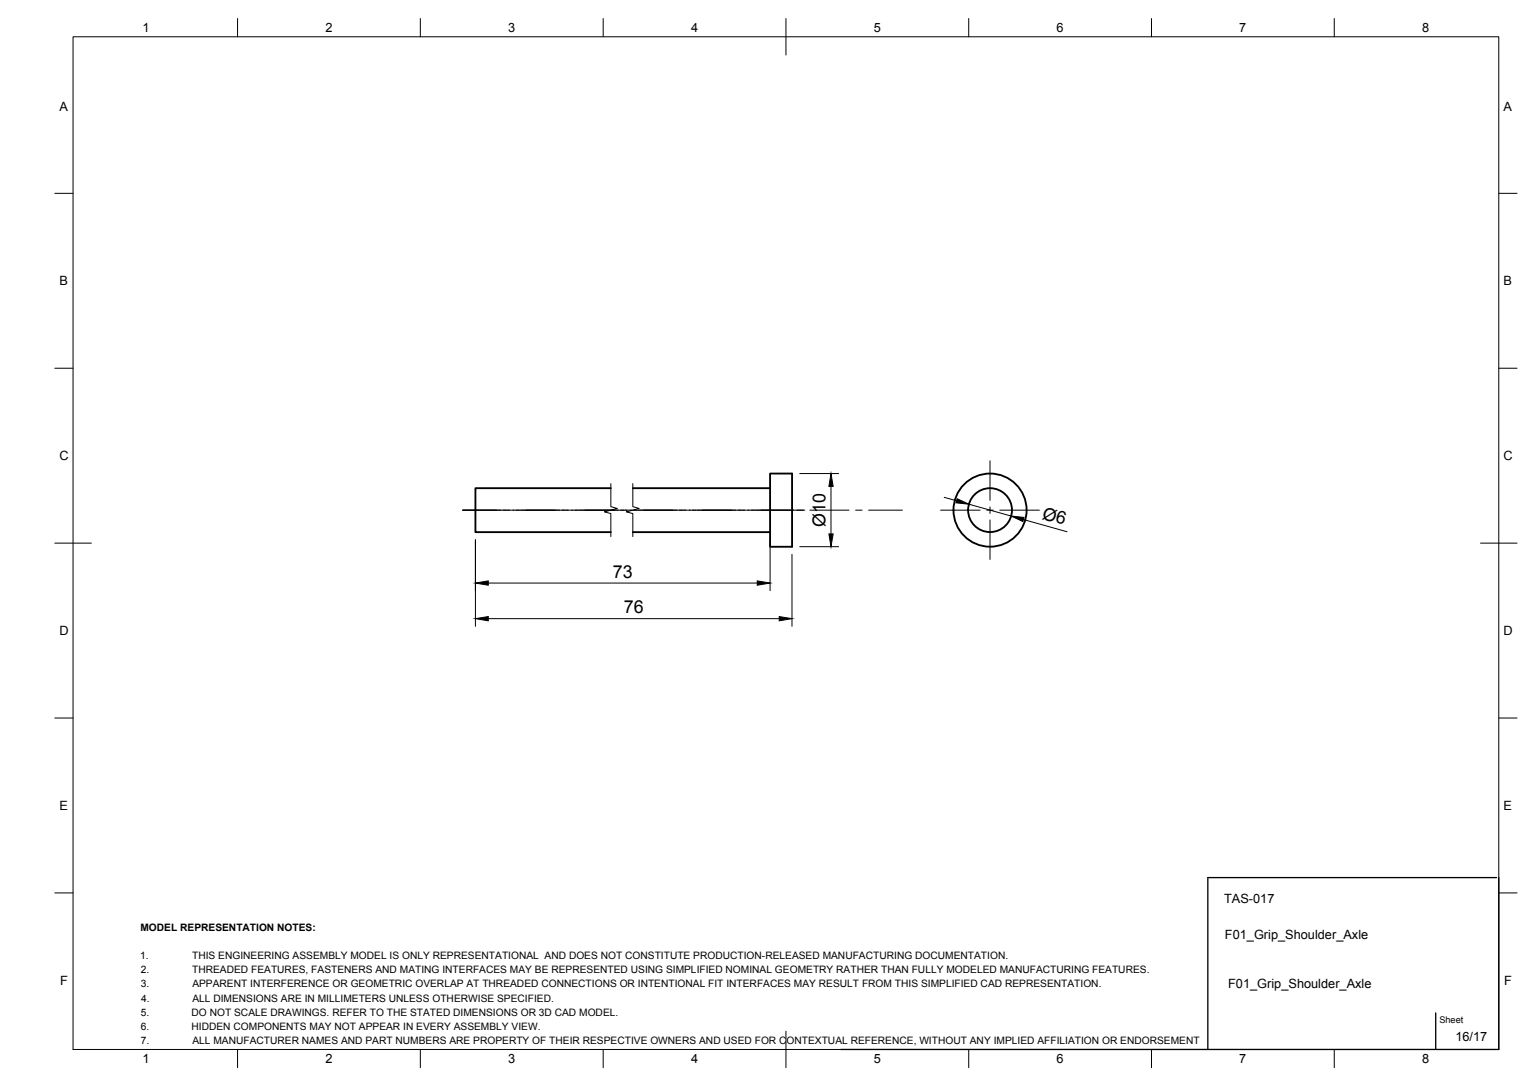
ISO-10303-21;
HEADER;
/* Generated by software containing ST-Developer
 * from STEP Tools, Inc. (www.steptools.com) 
 */

FILE_DESCRIPTION(
/* description */ ('STEP AP203'),
/* implementation_level */ '2;1');

FILE_NAME(
/* name */ 'F01_Grip_Shoulder_Axle.step',
/* time_stamp */ '2026-11-15T15:04:01-08:00',
/* author */ (''),
/* organization */ (''),
/* preprocessor_version */ 'ST-DEVELOPER v20.2',
/* originating_system */ 'Autodesk Translation Framework v15.17.0.0',
/* authorisation */ '');

FILE_SCHEMA (('AUTOMOTIVE_DESIGN { 1 0 10303 214 3 1 1 }'));
ENDSEC;

DATA;
#10=MECHANICAL_DESIGN_GEOMETRIC_PRESENTATION_REPRESENTATION('',(#301),#16598);
#223=SHAPE_REPRESENTATION_RELATIONSHIP('SRR','None',#16717,#247);
#247=ADVANCED_BREP_SHAPE_REPRESENTATION('',(#271),#16593);
#271=MANIFOLD_SOLID_BREP('Body1',#9806);
#301=STYLED_ITEM('',(#16829),#271);
#421=FACE_BOUND('',#2085,.T.);
#871=PLANE('',#10822);
#872=PLANE('',#10823);
#873=PLANE('',#10824);
#1414=FACE_OUTER_BOUND('',#2080,.T.);
#1415=FACE_OUTER_BOUND('',#2081,.T.);
#1416=FACE_OUTER_BOUND('',#2082,.T.);
#1417=FACE_OUTER_BOUND('',#2083,.T.);
#1418=FACE_OUTER_BOUND('',#2084,.T.);
#2080=EDGE_LOOP('',(#8977,#8978,#8979,#8980));
#2081=EDGE_LOOP('',(#8981,#8982,#8983,#8984));
#2082=EDGE_LOOP('',(#8985));
#2083=EDGE_LOOP('',(#8986));
#2084=EDGE_LOOP('',(#8987));
#2085=EDGE_LOOP('',(#8988));
#3104=LINE('',#16295,#4152);
#3105=LINE('',#16301,#4153);
#4152=VECTOR('',#13380,5.);
#4153=VECTOR('',#13387,3.);
#4439=CIRCLE('',#10817,5.);
#4440=CIRCLE('',#10818,5.);
#4441=CIRCLE('',#10820,3.);
#4442=CIRCLE('',#10821,3.);
#5247=VERTEX_POINT('',#16292);
#5248=VERTEX_POINT('',#16294);
#5249=VERTEX_POINT('',#16298);
#5250=VERTEX_POINT('',#16300);
#6501=EDGE_CURVE('',#5247,#5247,#4439,.T.);
#6502=EDGE_CURVE('',#5247,#5248,#3104,.T.);
#6503=EDGE_CURVE('',#5248,#5248,#4440,.T.);
#6504=EDGE_CURVE('',#5249,#5249,#4441,.T.);
#6505=EDGE_CURVE('',#5249,#5250,#3105,.T.);
#6506=EDGE_CURVE('',#5250,#5250,#4442,.T.);
#8977=ORIENTED_EDGE('',*,*,#6501,.T.);
#8978=ORIENTED_EDGE('',*,*,#6502,.T.);
#8979=ORIENTED_EDGE('',*,*,#6503,.F.);
#8980=ORIENTED_EDGE('',*,*,#6502,.F.);
#8981=ORIENTED_EDGE('',*,*,#6504,.T.);
#8982=ORIENTED_EDGE('',*,*,#6505,.T.);
#8983=ORIENTED_EDGE('',*,*,#6506,.F.);
#8984=ORIENTED_EDGE('',*,*,#6505,.F.);
#8985=ORIENTED_EDGE('',*,*,#6504,.F.);
#8986=ORIENTED_EDGE('',*,*,#6503,.T.);
#8987=ORIENTED_EDGE('',*,*,#6501,.F.);
#8988=ORIENTED_EDGE('',*,*,#6506,.T.);
#9228=CYLINDRICAL_SURFACE('',#10816,5.);
#9229=CYLINDRICAL_SURFACE('',#10819,3.);
#9739=ADVANCED_FACE('',(#1414),#9228,.T.);
#9740=ADVANCED_FACE('',(#1415),#9229,.T.);
#9741=ADVANCED_FACE('',(#1416),#871,.F.);
#9742=ADVANCED_FACE('',(#1417),#872,.T.);
#9743=ADVANCED_FACE('',(#1418,#421),#873,.F.);
#9806=CLOSED_SHELL('',(#9739,#9740,#9741,#9742,#9743));
#10815=AXIS2_PLACEMENT_3D('',#16290,#13374,#13375);
#10816=AXIS2_PLACEMENT_3D('',#16291,#13376,#13377);
#10817=AXIS2_PLACEMENT_3D('',#16293,#13378,#13379);
#10818=AXIS2_PLACEMENT_3D('',#16296,#13381,#13382);
#10819=AXIS2_PLACEMENT_3D('',#16297,#13383,#13384);
#10820=AXIS2_PLACEMENT_3D('',#16299,#13385,#13386);
#10821=AXIS2_PLACEMENT_3D('',#16302,#13388,#13389);
#10822=AXIS2_PLACEMENT_3D('',#16303,#13390,#13391);
#10823=AXIS2_PLACEMENT_3D('',#16304,#13392,#13393);
#10824=AXIS2_PLACEMENT_3D('',#16305,#13394,#13395);
#13374=DIRECTION('axis',(0.,0.,1.));
#13375=DIRECTION('refdir',(1.,0.,0.));
#13376=DIRECTION('center_axis',(0.,0.,-1.));
#13377=DIRECTION('ref_axis',(-1.,0.,0.));
#13378=DIRECTION('center_axis',(0.,0.,1.));
#13379=DIRECTION('ref_axis',(1.,0.,0.));
#13380=DIRECTION('',(0.,0.,1.));
#13381=DIRECTION('center_axis',(0.,0.,1.));
#13382=DIRECTION('ref_axis',(1.,0.,0.));
#13383=DIRECTION('center_axis',(0.,0.,-1.));
#13384=DIRECTION('ref_axis',(-1.,0.,0.));
#13385=DIRECTION('center_axis',(0.,0.,1.));
#13386=DIRECTION('ref_axis',(1.,0.,0.));
#13387=DIRECTION('',(0.,0.,1.));
#13388=DIRECTION('center_axis',(0.,0.,1.));
#13389=DIRECTION('ref_axis',(1.,0.,0.));
#13390=DIRECTION('center_axis',(0.,0.,1.));
#13391=DIRECTION('ref_axis',(1.,0.,0.));
#13392=DIRECTION('center_axis',(0.,0.,1.));
#13393=DIRECTION('ref_axis',(1.,0.,0.));
#13394=DIRECTION('center_axis',(0.,0.,1.));
#13395=DIRECTION('ref_axis',(1.,0.,0.));
#16290=CARTESIAN_POINT('',(0.,0.,0.));
#16291=CARTESIAN_POINT('Origin',(0.,0.,76.));
#16292=CARTESIAN_POINT('',(5.,-6.12323399573677E-16,73.));
#16293=CARTESIAN_POINT('Origin',(0.,0.,73.));
#16294=CARTESIAN_POINT('',(5.,-6.12323399573677E-16,76.));
#16295=CARTESIAN_POINT('',(5.,-6.12323399573677E-16,76.));
#16296=CARTESIAN_POINT('Origin',(0.,0.,76.));
#16297=CARTESIAN_POINT('Origin',(0.,0.,73.));
#16298=CARTESIAN_POINT('',(3.,-3.67394039744206E-16,0.));
#16299=CARTESIAN_POINT('Origin',(0.,0.,0.));
#16300=CARTESIAN_POINT('',(3.,-3.67394039744206E-16,73.));
#16301=CARTESIAN_POINT('',(3.,-3.67394039744206E-16,73.));
#16302=CARTESIAN_POINT('Origin',(0.,0.,73.));
#16303=CARTESIAN_POINT('Origin',(0.,0.,0.));
#16304=CARTESIAN_POINT('Origin',(0.,0.,76.));
#16305=CARTESIAN_POINT('Origin',(0.,0.,73.));
#16567=UNCERTAINTY_MEASURE_WITH_UNIT(LENGTH_MEASURE(0.01),#16599,
'DISTANCE_ACCURACY_VALUE',
'Maximum model space distance between geometric entities at asserted c
onnectivities');
#16572=UNCERTAINTY_MEASURE_WITH_UNIT(LENGTH_MEASURE(0.01),#16599,
'DISTANCE_ACCURACY_VALUE',
'Maximum model space distance between geometric entities at asserted c
onnectivities');
#16593=(
GEOMETRIC_REPRESENTATION_CONTEXT(3)
GLOBAL_UNCERTAINTY_ASSIGNED_CONTEXT((#16567))
GLOBAL_UNIT_ASSIGNED_CONTEXT((#16599,#16601,#16602))
REPRESENTATION_CONTEXT('','3D')
);
#16598=(
GEOMETRIC_REPRESENTATION_CONTEXT(3)
GLOBAL_UNCERTAINTY_ASSIGNED_CONTEXT((#16572))
GLOBAL_UNIT_ASSIGNED_CONTEXT((#16599,#16601,#16602))
REPRESENTATION_CONTEXT('','3D')
);
#16599=(
LENGTH_UNIT()
NAMED_UNIT(*)
SI_UNIT(.MILLI.,.METRE.)
);
#16601=(
NAMED_UNIT(*)
PLANE_ANGLE_UNIT()
SI_UNIT($,.RADIAN.)
);
#16602=(
NAMED_UNIT(*)
SI_UNIT($,.STERADIAN.)
SOLID_ANGLE_UNIT()
);
#16623=SHAPE_DEFINITION_REPRESENTATION(#16648,#16717);
#16648=PRODUCT_DEFINITION_SHAPE('',$,#16743);
#16717=SHAPE_REPRESENTATION('',(#10815),#16593);
#16722=PRODUCT_DEFINITION_CONTEXT('part definition',#16799,'design');
#16743=PRODUCT_DEFINITION('F01_Grip_Shoulder_Axle',
'F01_Grip_Shoulder_Axle',#16768,#16722);
#16768=PRODUCT_DEFINITION_FORMATION('',$,#16821);
#16799=APPLICATION_CONTEXT(
'Core Data for Automotive Mechanical Design Process');
#16800=PRODUCT_CONTEXT('part definition',#16799,'mechanical');
#16821=PRODUCT('F01_Grip_Shoulder_Axle','F01_Grip_Shoulder_Axle',$,(#16800));
#16829=PRESENTATION_STYLE_ASSIGNMENT((#16838));
#16838=SURFACE_STYLE_USAGE(.BOTH.,#16847);
#16847=SURFACE_SIDE_STYLE('',(#16856));
#16856=SURFACE_STYLE_FILL_AREA(#16865);
#16865=FILL_AREA_STYLE('Light Gray',(#16874));
#16874=FILL_AREA_STYLE_COLOUR('Light Gray',#16883);
#16883=COLOUR_RGB('Light Gray',0.827450980392157,0.827450980392157,0.827450980392157);
ENDSEC;
END-ISO-10303-21;
